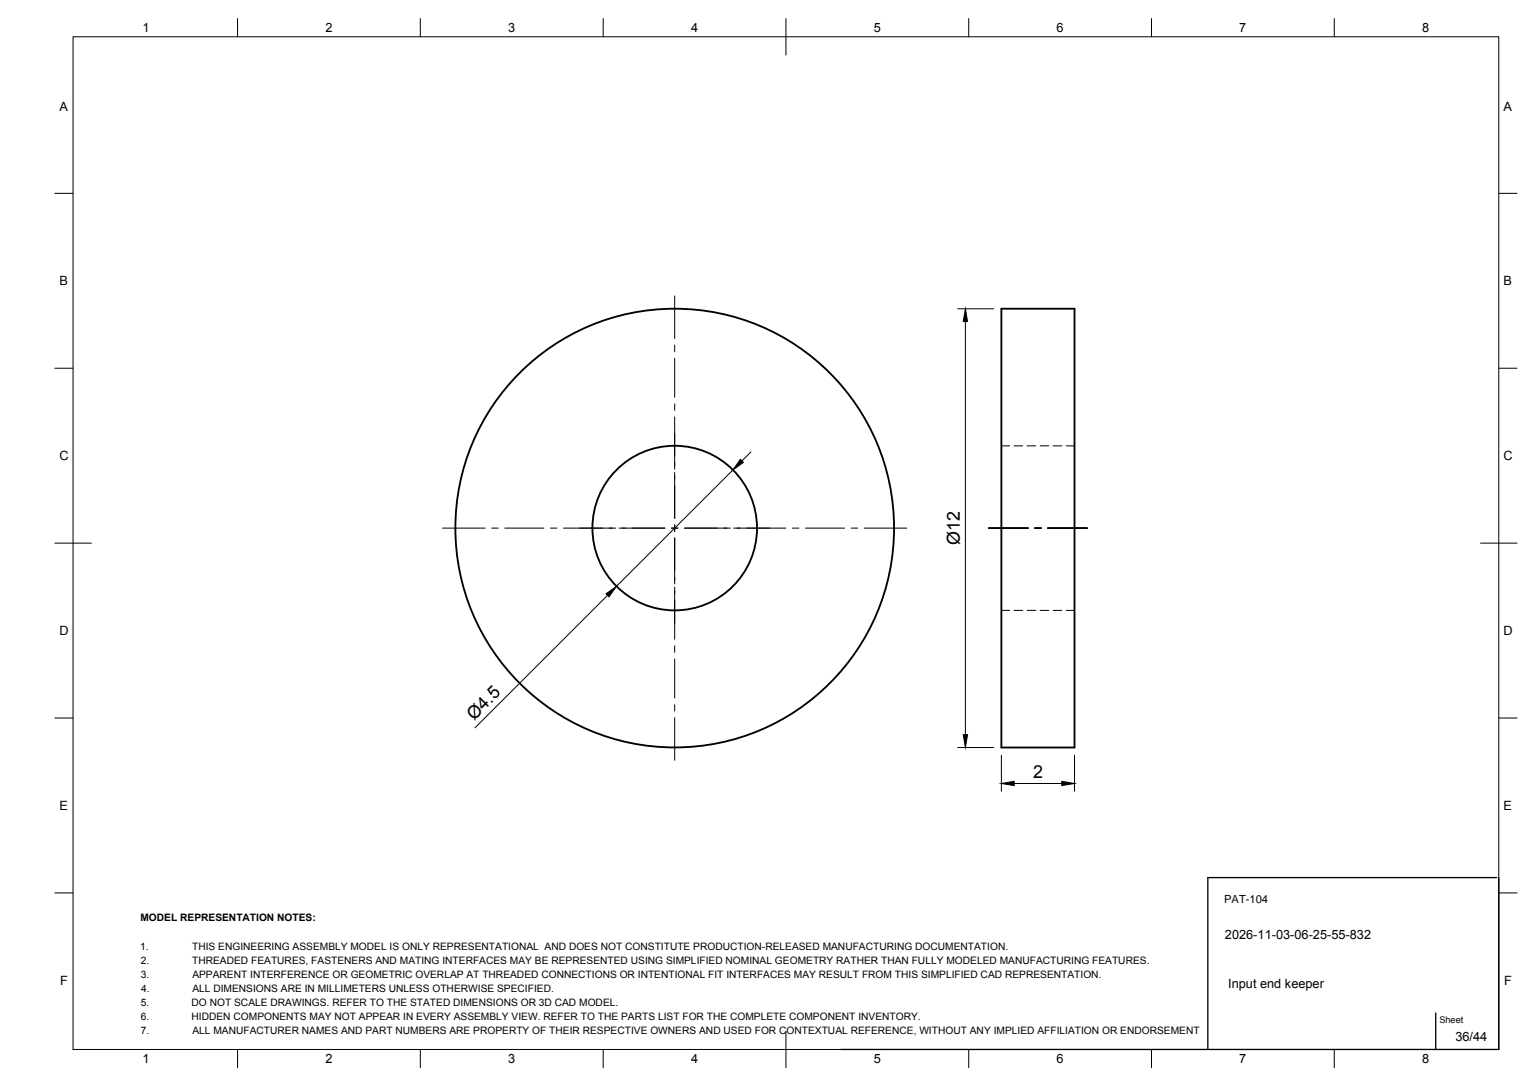
ISO-10303-21;
HEADER;
/* Generated by software containing ST-Developer
 * from STEP Tools, Inc. (www.steptools.com) 
 */

FILE_DESCRIPTION(
/* description */ ('Timing belt drive module 2 mm Pitch Timing 20T-40T'),

/* implementation_level */ '2;1');

FILE_NAME(
/* name */ 'Input end keeper.step',
/* time_stamp */ '2026-10-28T03:25:12-07:00',
/* author */ (''),
/* organization */ (''),
/* preprocessor_version */ 'ST-DEVELOPER v20.2',
/* originating_system */ 'Autodesk Translation Framework v15.17.0.0',
/* authorisation */ '');

FILE_SCHEMA (('AUTOMOTIVE_DESIGN { 1 0 10303 214 3 1 1 }'));
ENDSEC;

DATA;
#10=MECHANICAL_DESIGN_GEOMETRIC_PRESENTATION_REPRESENTATION('',(#572),#17830);
#471=SHAPE_REPRESENTATION_RELATIONSHIP('SRR','None',#18044,#514);
#514=ADVANCED_BREP_SHAPE_REPRESENTATION('',(#628),#17819);
#572=STYLED_ITEM('',(#18310),#628);
#628=MANIFOLD_SOLID_BREP('Body1',#9031);
#739=FACE_BOUND('',#1915,.T.);
#740=FACE_BOUND('',#1917,.T.);
#924=PLANE('',#10256);
#925=PLANE('',#10257);
#1289=FACE_OUTER_BOUND('',#1912,.T.);
#1290=FACE_OUTER_BOUND('',#1913,.T.);
#1291=FACE_OUTER_BOUND('',#1914,.T.);
#1292=FACE_OUTER_BOUND('',#1916,.T.);
#1912=EDGE_LOOP('',(#7153,#7154,#7155,#7156));
#1913=EDGE_LOOP('',(#7157,#7158,#7159,#7160));
#1914=EDGE_LOOP('',(#7161));
#1915=EDGE_LOOP('',(#7162));
#1916=EDGE_LOOP('',(#7163));
#1917=EDGE_LOOP('',(#7164));
#2498=CIRCLE('',#10251,0.225);
#2499=CIRCLE('',#10252,0.225);
#2500=CIRCLE('',#10254,0.6);
#2501=CIRCLE('',#10255,0.6);
#3090=LINE('',#16050,#3568);
#3091=LINE('',#16056,#3569);
#3568=VECTOR('',#12581,0.225);
#3569=VECTOR('',#12588,0.6);
#4221=VERTEX_POINT('',#16047);
#4222=VERTEX_POINT('',#16049);
#4223=VERTEX_POINT('',#16053);
#4224=VERTEX_POINT('',#16055);
#5259=EDGE_CURVE('',#4221,#4221,#2498,.T.);
#5260=EDGE_CURVE('',#4221,#4222,#3090,.T.);
#5261=EDGE_CURVE('',#4222,#4222,#2499,.T.);
#5262=EDGE_CURVE('',#4223,#4223,#2500,.T.);
#5263=EDGE_CURVE('',#4223,#4224,#3091,.T.);
#5264=EDGE_CURVE('',#4224,#4224,#2501,.T.);
#7153=ORIENTED_EDGE('',*,*,#5259,.F.);
#7154=ORIENTED_EDGE('',*,*,#5260,.T.);
#7155=ORIENTED_EDGE('',*,*,#5261,.T.);
#7156=ORIENTED_EDGE('',*,*,#5260,.F.);
#7157=ORIENTED_EDGE('',*,*,#5262,.F.);
#7158=ORIENTED_EDGE('',*,*,#5263,.T.);
#7159=ORIENTED_EDGE('',*,*,#5264,.T.);
#7160=ORIENTED_EDGE('',*,*,#5263,.F.);
#7161=ORIENTED_EDGE('',*,*,#5262,.T.);
#7162=ORIENTED_EDGE('',*,*,#5259,.T.);
#7163=ORIENTED_EDGE('',*,*,#5264,.F.);
#7164=ORIENTED_EDGE('',*,*,#5261,.F.);
#8308=CYLINDRICAL_SURFACE('',#10250,0.225);
#8309=CYLINDRICAL_SURFACE('',#10253,0.6);
#8787=ADVANCED_FACE('',(#1289),#8308,.F.);
#8788=ADVANCED_FACE('',(#1290),#8309,.T.);
#8789=ADVANCED_FACE('',(#1291,#739),#924,.T.);
#8790=ADVANCED_FACE('',(#1292,#740),#925,.F.);
#9031=CLOSED_SHELL('',(#8787,#8788,#8789,#8790));
#10249=AXIS2_PLACEMENT_3D('',#16045,#12575,#12576);
#10250=AXIS2_PLACEMENT_3D('',#16046,#12577,#12578);
#10251=AXIS2_PLACEMENT_3D('',#16048,#12579,#12580);
#10252=AXIS2_PLACEMENT_3D('',#16051,#12582,#12583);
#10253=AXIS2_PLACEMENT_3D('',#16052,#12584,#12585);
#10254=AXIS2_PLACEMENT_3D('',#16054,#12586,#12587);
#10255=AXIS2_PLACEMENT_3D('',#16057,#12589,#12590);
#10256=AXIS2_PLACEMENT_3D('',#16058,#12591,#12592);
#10257=AXIS2_PLACEMENT_3D('',#16059,#12593,#12594);
#12575=DIRECTION('axis',(0.,0.,1.));
#12576=DIRECTION('refdir',(1.,0.,0.));
#12577=DIRECTION('center_axis',(0.,1.,0.));
#12578=DIRECTION('ref_axis',(1.,0.,0.));
#12579=DIRECTION('center_axis',(0.,-1.,0.));
#12580=DIRECTION('ref_axis',(1.,0.,0.));
#12581=DIRECTION('',(0.,-1.,0.));
#12582=DIRECTION('center_axis',(0.,-1.,0.));
#12583=DIRECTION('ref_axis',(1.,0.,0.));
#12584=DIRECTION('center_axis',(0.,1.,0.));
#12585=DIRECTION('ref_axis',(1.,0.,0.));
#12586=DIRECTION('center_axis',(0.,1.,0.));
#12587=DIRECTION('ref_axis',(1.,0.,0.));
#12588=DIRECTION('',(0.,-1.,0.));
#12589=DIRECTION('center_axis',(0.,1.,0.));
#12590=DIRECTION('ref_axis',(1.,0.,0.));
#12591=DIRECTION('center_axis',(0.,1.,0.));
#12592=DIRECTION('ref_axis',(1.,0.,0.));
#12593=DIRECTION('center_axis',(0.,1.,0.));
#12594=DIRECTION('ref_axis',(1.,0.,0.));
#16045=CARTESIAN_POINT('',(0.,0.,0.));
#16046=CARTESIAN_POINT('Origin',(0.,-5.2,7.));
#16047=CARTESIAN_POINT('',(-0.225,-5.,7.));
#16048=CARTESIAN_POINT('Origin',(0.,-5.,7.));
#16049=CARTESIAN_POINT('',(-0.225,-5.2,7.));
#16050=CARTESIAN_POINT('',(-0.225,-5.2,7.));
#16051=CARTESIAN_POINT('Origin',(0.,-5.2,7.));
#16052=CARTESIAN_POINT('Origin',(0.,-5.2,7.));
#16053=CARTESIAN_POINT('',(-0.6,-5.,7.));
#16054=CARTESIAN_POINT('Origin',(0.,-5.,7.));
#16055=CARTESIAN_POINT('',(-0.6,-5.2,7.));
#16056=CARTESIAN_POINT('',(-0.6,-5.2,7.));
#16057=CARTESIAN_POINT('Origin',(0.,-5.2,7.));
#16058=CARTESIAN_POINT('Origin',(0.,-5.,7.));
#16059=CARTESIAN_POINT('Origin',(0.,-5.2,7.));
#17769=UNCERTAINTY_MEASURE_WITH_UNIT(LENGTH_MEASURE(0.001),#17831,
'DISTANCE_ACCURACY_VALUE',
'Maximum model space distance between geometric entities at asserted c
onnectivities');
#17780=UNCERTAINTY_MEASURE_WITH_UNIT(LENGTH_MEASURE(0.001),#17831,
'DISTANCE_ACCURACY_VALUE',
'Maximum model space distance between geometric entities at asserted c
onnectivities');
#17819=(
GEOMETRIC_REPRESENTATION_CONTEXT(3)
GLOBAL_UNCERTAINTY_ASSIGNED_CONTEXT((#17769))
GLOBAL_UNIT_ASSIGNED_CONTEXT((#17831,#17833,#17834))
REPRESENTATION_CONTEXT('','3D')
);
#17830=(
GEOMETRIC_REPRESENTATION_CONTEXT(3)
GLOBAL_UNCERTAINTY_ASSIGNED_CONTEXT((#17780))
GLOBAL_UNIT_ASSIGNED_CONTEXT((#17831,#17833,#17834))
REPRESENTATION_CONTEXT('','3D')
);
#17831=(
LENGTH_UNIT()
NAMED_UNIT(*)
SI_UNIT(.CENTI.,.METRE.)
);
#17833=(
NAMED_UNIT(*)
PLANE_ANGLE_UNIT()
SI_UNIT($,.RADIAN.)
);
#17834=(
NAMED_UNIT(*)
SI_UNIT($,.STERADIAN.)
SOLID_ANGLE_UNIT()
);
#17873=SHAPE_DEFINITION_REPRESENTATION(#17932,#18044);
#17932=PRODUCT_DEFINITION_SHAPE('',$,#18094);
#18044=SHAPE_REPRESENTATION('',(#10249),#17819);
#18055=PRODUCT_DEFINITION_CONTEXT('part definition',#18204,'design');
#18094=PRODUCT_DEFINITION('Input end keeper','Input end keeper',#18143,
#18055);
#18143=PRODUCT_DEFINITION_FORMATION('',$,#18244);
#18204=APPLICATION_CONTEXT(
'Core Data for Automotive Mechanical Design Process');
#18205=PRODUCT_CONTEXT('part definition',#18204,'mechanical');
#18244=PRODUCT('Input end keeper','Input end keeper','Input end keeper',
(#18205));
#18304=COLOUR_RGB('Sky Blue',0.24,0.69,0.87);
#18305=FILL_AREA_STYLE_COLOUR('',#18304);
#18306=FILL_AREA_STYLE('',(#18305));
#18307=SURFACE_STYLE_FILL_AREA(#18306);
#18308=SURFACE_SIDE_STYLE('',(#18307));
#18309=SURFACE_STYLE_USAGE(.BOTH.,#18308);
#18310=PRESENTATION_STYLE_ASSIGNMENT((#18309));
ENDSEC;
END-ISO-10303-21;
